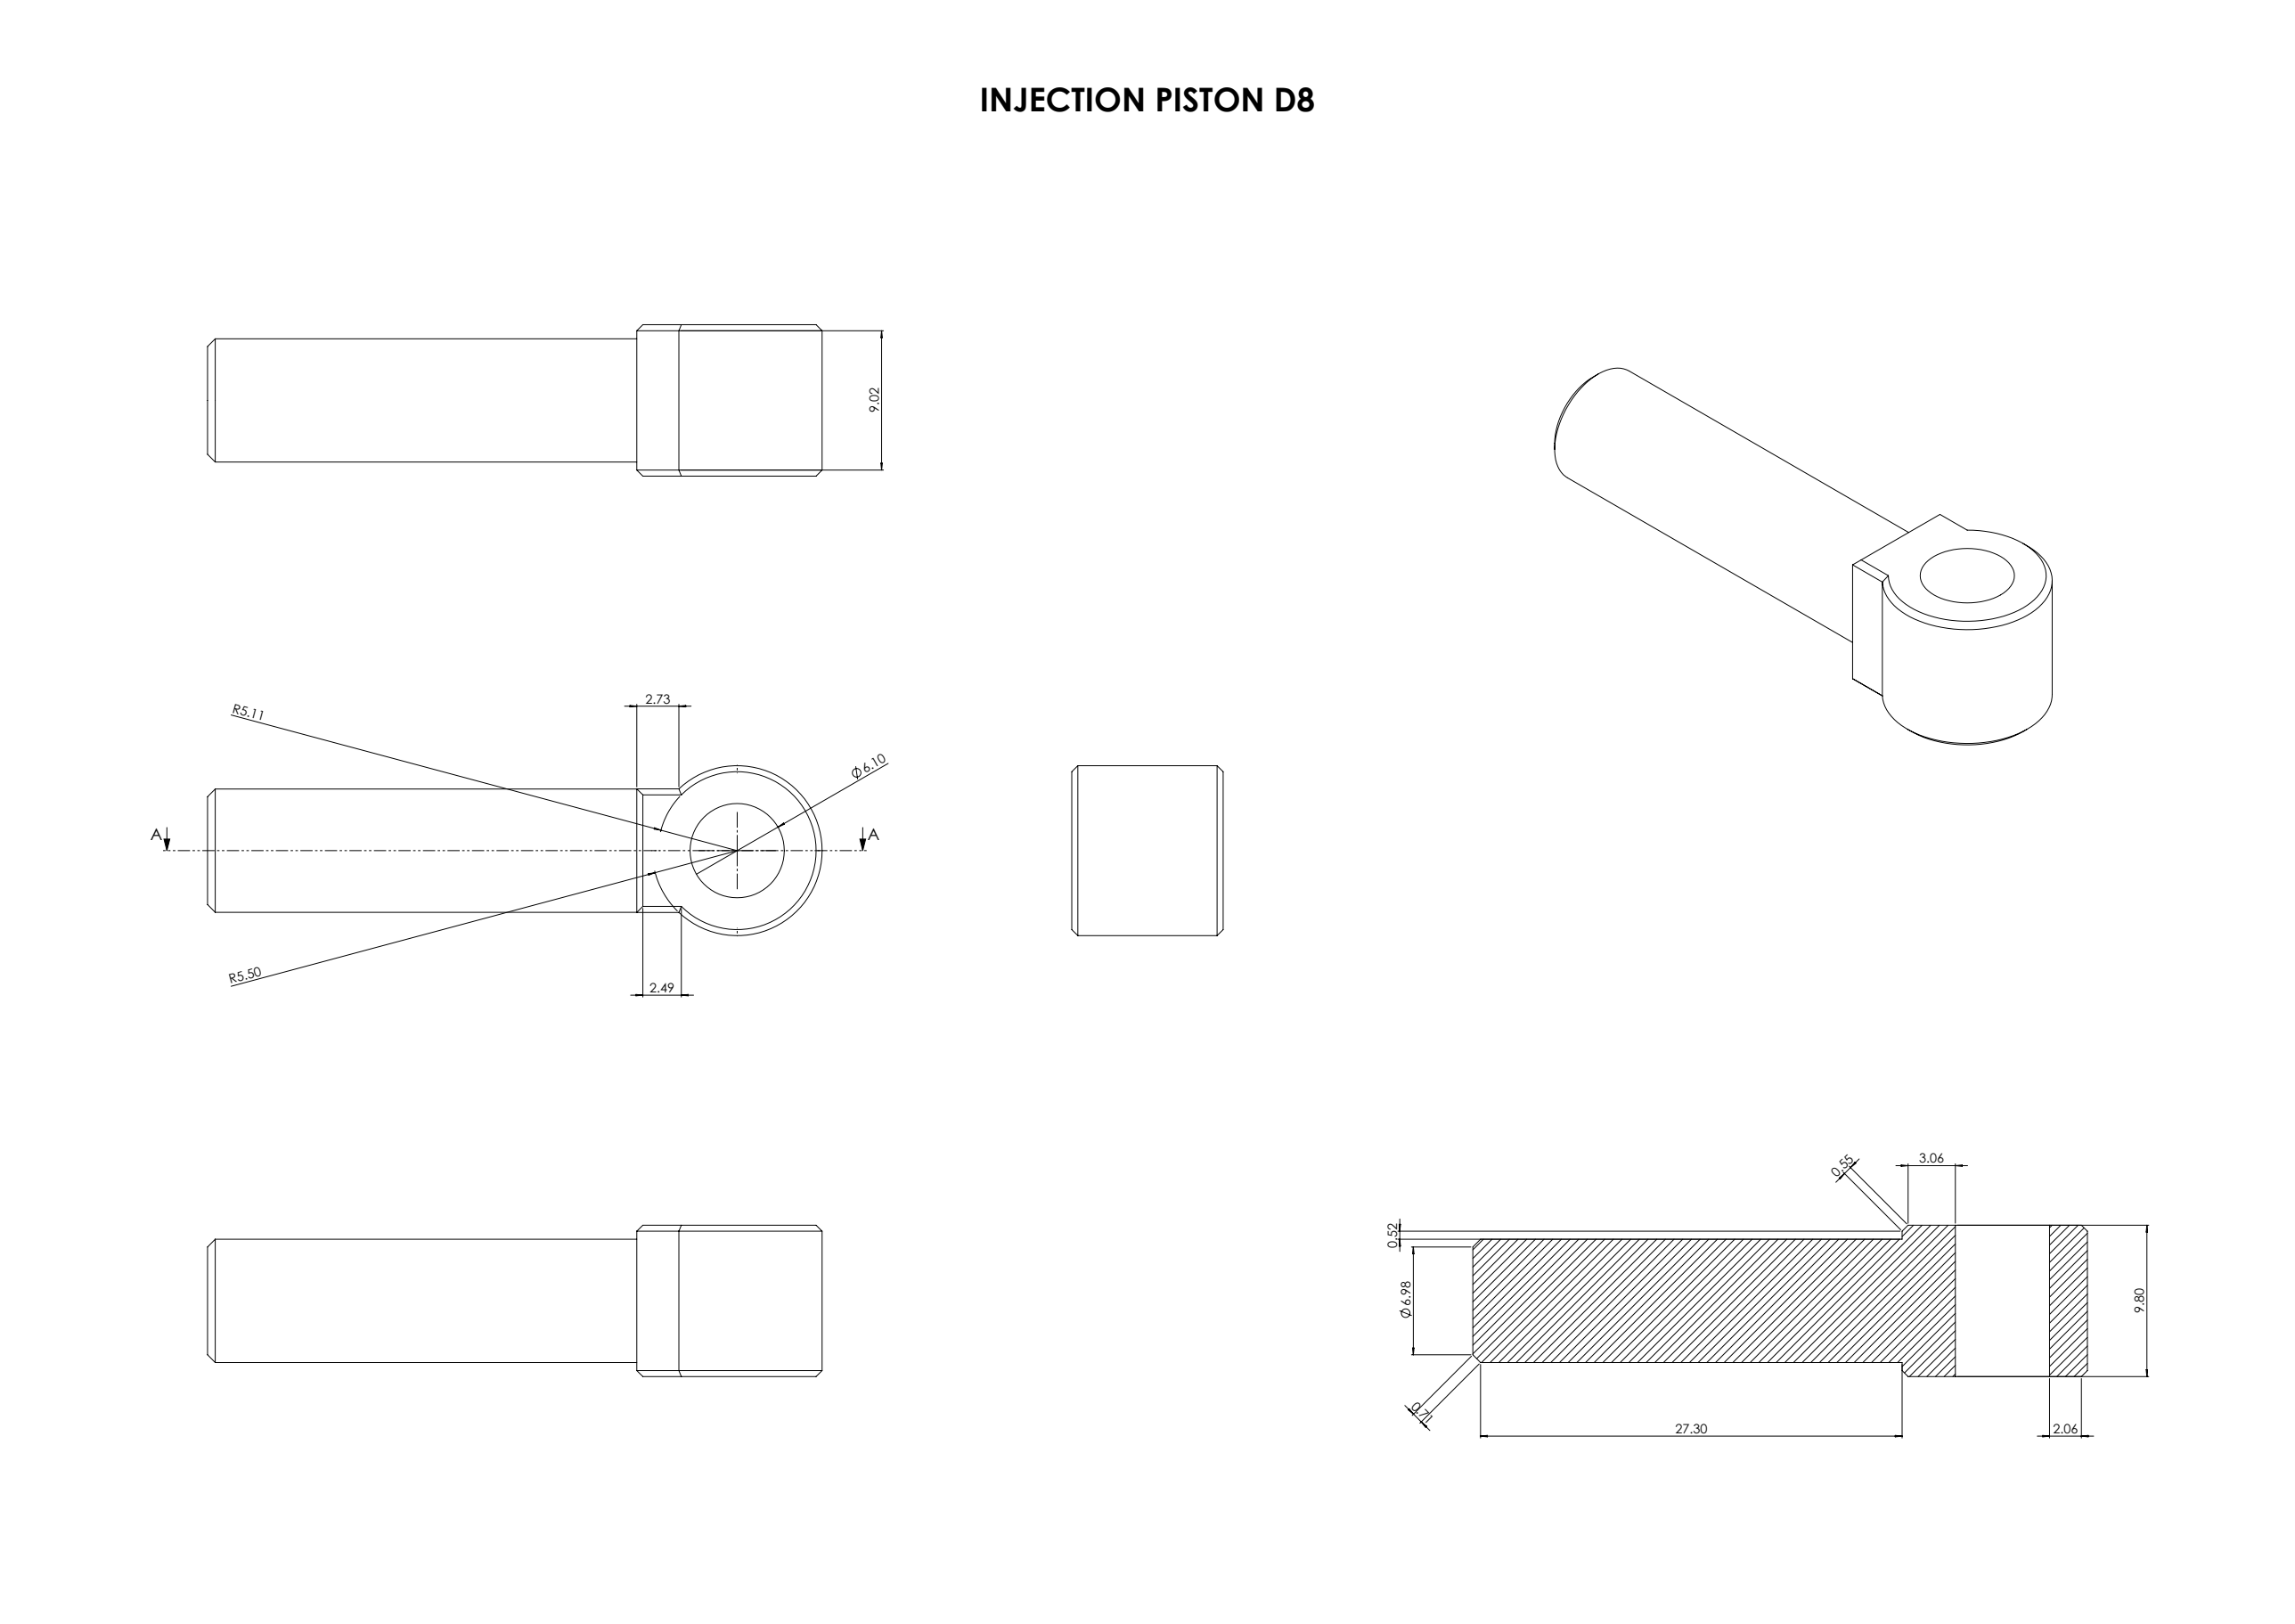
ISO-10303-21;
HEADER;
/* Generated by software containing ST-Developer
 * from STEP Tools, Inc. (www.steptools.com) 
 */

FILE_DESCRIPTION(
/* description */ (''),
/* implementation_level */ '2;1');

FILE_NAME(
/* name */ '13_Injection_Piston_D8.step',
/* time_stamp */ '2026-10-26T03:55:20-07:00',
/* author */ (''),
/* organization */ (''),
/* preprocessor_version */ 'ST-DEVELOPER v20.2',
/* originating_system */ 'Autodesk Translation Framework v15.15.0.0',
/* authorisation */ '');

FILE_SCHEMA (('AUTOMOTIVE_DESIGN { 1 0 10303 214 3 1 1 }'));
ENDSEC;

DATA;
#10=MECHANICAL_DESIGN_GEOMETRIC_PRESENTATION_REPRESENTATION('',(#193),#45236);
#153=SHAPE_REPRESENTATION_RELATIONSHIP('SRR','None',#45332,#173);
#173=ADVANCED_BREP_SHAPE_REPRESENTATION('',(#213),#45234);
#193=STYLED_ITEM('',(#45477),#213);
#213=MANIFOLD_SOLID_BREP('Body1',#16535);
#810=B_SPLINE_CURVE_WITH_KNOTS('',3,(#45054,#45055,#45056,#45057),
 .UNSPECIFIED.,.F.,.F.,(4,4),(-0.0573534079505418,0.),.UNSPECIFIED.);
#811=B_SPLINE_CURVE_WITH_KNOTS('',3,(#45060,#45061,#45062,#45063),
 .UNSPECIFIED.,.F.,.F.,(4,4),(-0.0573534079505118,0.),.UNSPECIFIED.);
#812=B_SPLINE_CURVE_WITH_KNOTS('',3,(#45094,#45095,#45096,#45097),
 .UNSPECIFIED.,.F.,.F.,(4,4),(-0.0573537350950076,0.),.UNSPECIFIED.);
#813=B_SPLINE_CURVE_WITH_KNOTS('',3,(#45100,#45101,#45102,#45103),
 .UNSPECIFIED.,.F.,.F.,(4,4),(-0.0573534079504966,0.),.UNSPECIFIED.);
#1059=FACE_BOUND('',#3866,.T.);
#1060=FACE_BOUND('',#3873,.T.);
#1061=FACE_BOUND('',#3876,.T.);
#1547=PLANE('',#18058);
#1548=PLANE('',#18059);
#1549=PLANE('',#18060);
#1550=PLANE('',#18061);
#1551=PLANE('',#18064);
#1552=PLANE('',#18068);
#1553=PLANE('',#18069);
#1554=PLANE('',#18070);
#1555=PLANE('',#18071);
#1556=PLANE('',#18072);
#1557=PLANE('',#18075);
#1558=PLANE('',#18077);
#1810=CYLINDRICAL_SURFACE('',#18062,5.5);
#1811=CYLINDRICAL_SURFACE('',#18074,3.05);
#1812=CYLINDRICAL_SURFACE('',#18081,3.99);
#2765=FACE_OUTER_BOUND('',#3859,.T.);
#2766=FACE_OUTER_BOUND('',#3860,.T.);
#2767=FACE_OUTER_BOUND('',#3861,.T.);
#2768=FACE_OUTER_BOUND('',#3862,.T.);
#2769=FACE_OUTER_BOUND('',#3863,.T.);
#2770=FACE_OUTER_BOUND('',#3864,.T.);
#2771=FACE_OUTER_BOUND('',#3865,.T.);
#2772=FACE_OUTER_BOUND('',#3867,.T.);
#2773=FACE_OUTER_BOUND('',#3868,.T.);
#2774=FACE_OUTER_BOUND('',#3869,.T.);
#2775=FACE_OUTER_BOUND('',#3870,.T.);
#2776=FACE_OUTER_BOUND('',#3871,.T.);
#2777=FACE_OUTER_BOUND('',#3872,.T.);
#2778=FACE_OUTER_BOUND('',#3874,.T.);
#2779=FACE_OUTER_BOUND('',#3875,.T.);
#2780=FACE_OUTER_BOUND('',#3877,.T.);
#2781=FACE_OUTER_BOUND('',#3878,.T.);
#2782=FACE_OUTER_BOUND('',#3879,.T.);
#3859=EDGE_LOOP('',(#15382,#15383,#15384,#15385));
#3860=EDGE_LOOP('',(#15386,#15387,#15388,#15389));
#3861=EDGE_LOOP('',(#15390,#15391,#15392,#15393));
#3862=EDGE_LOOP('',(#15394,#15395,#15396,#15397));
#3863=EDGE_LOOP('',(#15398,#15399,#15400,#15401));
#3864=EDGE_LOOP('',(#15402,#15403,#15404,#15405));
#3865=EDGE_LOOP('',(#15406,#15407,#15408,#15409));
#3866=EDGE_LOOP('',(#15410));
#3867=EDGE_LOOP('',(#15411,#15412,#15413,#15414));
#3868=EDGE_LOOP('',(#15415,#15416,#15417,#15418));
#3869=EDGE_LOOP('',(#15419,#15420,#15421,#15422));
#3870=EDGE_LOOP('',(#15423,#15424,#15425,#15426));
#3871=EDGE_LOOP('',(#15427,#15428,#15429,#15430));
#3872=EDGE_LOOP('',(#15431,#15432,#15433,#15434));
#3873=EDGE_LOOP('',(#15435));
#3874=EDGE_LOOP('',(#15436,#15437,#15438,#15439));
#3875=EDGE_LOOP('',(#15440,#15441,#15442,#15443));
#3876=EDGE_LOOP('',(#15444));
#3877=EDGE_LOOP('',(#15445));
#3878=EDGE_LOOP('',(#15446,#15447,#15448,#15449));
#3879=EDGE_LOOP('',(#15450,#15451,#15452,#15453));
#5166=LINE('',#45066,#6477);
#5167=LINE('',#45068,#6478);
#5168=LINE('',#45069,#6479);
#5169=LINE('',#45072,#6480);
#5170=LINE('',#45074,#6481);
#5171=LINE('',#45075,#6482);
#5172=LINE('',#45077,#6483);
#5173=LINE('',#45078,#6484);
#5174=LINE('',#45081,#6485);
#5175=LINE('',#45083,#6486);
#5176=LINE('',#45084,#6487);
#5177=LINE('',#45087,#6488);
#5178=LINE('',#45106,#6489);
#5179=LINE('',#45107,#6490);
#5180=LINE('',#45110,#6491);
#5181=LINE('',#45112,#6492);
#5182=LINE('',#45113,#6493);
#5183=LINE('',#45115,#6494);
#5184=LINE('',#45116,#6495);
#5185=LINE('',#45118,#6496);
#5186=LINE('',#45123,#6497);
#5187=LINE('',#45133,#6498);
#5188=LINE('',#45135,#6499);
#6477=VECTOR('',#22005,10.);
#6478=VECTOR('',#22006,10.);
#6479=VECTOR('',#22007,10.);
#6480=VECTOR('',#22010,10.);
#6481=VECTOR('',#22011,10.);
#6482=VECTOR('',#22012,10.);
#6483=VECTOR('',#22015,10.);
#6484=VECTOR('',#22016,10.);
#6485=VECTOR('',#22019,10.);
#6486=VECTOR('',#22020,10.);
#6487=VECTOR('',#22021,10.);
#6488=VECTOR('',#22024,10.);
#6489=VECTOR('',#22037,10.);
#6490=VECTOR('',#22038,10.);
#6491=VECTOR('',#22041,10.);
#6492=VECTOR('',#22042,10.);
#6493=VECTOR('',#22043,10.);
#6494=VECTOR('',#22046,10.);
#6495=VECTOR('',#22047,10.);
#6496=VECTOR('',#22050,10.);
#6497=VECTOR('',#22057,3.05);
#6498=VECTOR('',#22070,3.74);
#6499=VECTOR('',#22073,3.99);
#6950=CIRCLE('',#18056,5.11);
#6951=CIRCLE('',#18057,5.5);
#6952=CIRCLE('',#18063,5.5);
#6953=CIRCLE('',#18065,3.05);
#6954=CIRCLE('',#18067,5.11);
#6955=CIRCLE('',#18073,3.05);
#6956=CIRCLE('',#18076,3.99);
#6957=CIRCLE('',#18078,3.49);
#6958=CIRCLE('',#18080,3.99);
#8435=VERTEX_POINT('',#45050);
#8436=VERTEX_POINT('',#45051);
#8437=VERTEX_POINT('',#45053);
#8438=VERTEX_POINT('',#45058);
#8439=VERTEX_POINT('',#45065);
#8440=VERTEX_POINT('',#45067);
#8441=VERTEX_POINT('',#45071);
#8442=VERTEX_POINT('',#45073);
#8443=VERTEX_POINT('',#45080);
#8444=VERTEX_POINT('',#45082);
#8445=VERTEX_POINT('',#45086);
#8446=VERTEX_POINT('',#45090);
#8447=VERTEX_POINT('',#45093);
#8448=VERTEX_POINT('',#45098);
#8449=VERTEX_POINT('',#45105);
#8450=VERTEX_POINT('',#45109);
#8451=VERTEX_POINT('',#45111);
#8452=VERTEX_POINT('',#45120);
#8453=VERTEX_POINT('',#45125);
#8454=VERTEX_POINT('',#45128);
#8455=VERTEX_POINT('',#45131);
#10754=EDGE_CURVE('',#8435,#8436,#6950,.T.);
#10755=EDGE_CURVE('',#8436,#8437,#810,.T.);
#10756=EDGE_CURVE('',#8437,#8438,#6951,.T.);
#10757=EDGE_CURVE('',#8435,#8438,#811,.T.);
#10758=EDGE_CURVE('',#8436,#8439,#5166,.T.);
#10759=EDGE_CURVE('',#8439,#8440,#5167,.T.);
#10760=EDGE_CURVE('',#8440,#8437,#5168,.T.);
#10761=EDGE_CURVE('',#8439,#8441,#5169,.T.);
#10762=EDGE_CURVE('',#8441,#8442,#5170,.T.);
#10763=EDGE_CURVE('',#8442,#8440,#5171,.T.);
#10764=EDGE_CURVE('',#8438,#8442,#5172,.T.);
#10765=EDGE_CURVE('',#8441,#8435,#5173,.T.);
#10766=EDGE_CURVE('',#8443,#8438,#5174,.T.);
#10767=EDGE_CURVE('',#8444,#8443,#5175,.T.);
#10768=EDGE_CURVE('',#8444,#8442,#5176,.T.);
#10769=EDGE_CURVE('',#8445,#8437,#5177,.T.);
#10770=EDGE_CURVE('',#8443,#8445,#6952,.T.);
#10771=EDGE_CURVE('',#8446,#8446,#6953,.T.);
#10772=EDGE_CURVE('',#8445,#8447,#812,.T.);
#10773=EDGE_CURVE('',#8447,#8448,#6954,.T.);
#10774=EDGE_CURVE('',#8448,#8443,#813,.T.);
#10775=EDGE_CURVE('',#8448,#8449,#5178,.T.);
#10776=EDGE_CURVE('',#8449,#8444,#5179,.T.);
#10777=EDGE_CURVE('',#8449,#8450,#5180,.T.);
#10778=EDGE_CURVE('',#8450,#8451,#5181,.T.);
#10779=EDGE_CURVE('',#8451,#8444,#5182,.T.);
#10780=EDGE_CURVE('',#8445,#8451,#5183,.T.);
#10781=EDGE_CURVE('',#8450,#8447,#5184,.T.);
#10782=EDGE_CURVE('',#8451,#8440,#5185,.T.);
#10783=EDGE_CURVE('',#8452,#8452,#6955,.T.);
#10784=EDGE_CURVE('',#8452,#8446,#5186,.T.);
#10785=EDGE_CURVE('',#8453,#8453,#6956,.T.);
#10786=EDGE_CURVE('',#8454,#8454,#6957,.T.);
#10787=EDGE_CURVE('',#8455,#8455,#6958,.T.);
#10788=EDGE_CURVE('',#8455,#8454,#5187,.T.);
#10789=EDGE_CURVE('',#8453,#8455,#5188,.T.);
#15382=ORIENTED_EDGE('',*,*,#10754,.T.);
#15383=ORIENTED_EDGE('',*,*,#10755,.T.);
#15384=ORIENTED_EDGE('',*,*,#10756,.T.);
#15385=ORIENTED_EDGE('',*,*,#10757,.F.);
#15386=ORIENTED_EDGE('',*,*,#10758,.T.);
#15387=ORIENTED_EDGE('',*,*,#10759,.T.);
#15388=ORIENTED_EDGE('',*,*,#10760,.T.);
#15389=ORIENTED_EDGE('',*,*,#10755,.F.);
#15390=ORIENTED_EDGE('',*,*,#10761,.T.);
#15391=ORIENTED_EDGE('',*,*,#10762,.T.);
#15392=ORIENTED_EDGE('',*,*,#10763,.T.);
#15393=ORIENTED_EDGE('',*,*,#10759,.F.);
#15394=ORIENTED_EDGE('',*,*,#10764,.T.);
#15395=ORIENTED_EDGE('',*,*,#10762,.F.);
#15396=ORIENTED_EDGE('',*,*,#10765,.T.);
#15397=ORIENTED_EDGE('',*,*,#10757,.T.);
#15398=ORIENTED_EDGE('',*,*,#10764,.F.);
#15399=ORIENTED_EDGE('',*,*,#10766,.F.);
#15400=ORIENTED_EDGE('',*,*,#10767,.F.);
#15401=ORIENTED_EDGE('',*,*,#10768,.T.);
#15402=ORIENTED_EDGE('',*,*,#10756,.F.);
#15403=ORIENTED_EDGE('',*,*,#10769,.F.);
#15404=ORIENTED_EDGE('',*,*,#10770,.F.);
#15405=ORIENTED_EDGE('',*,*,#10766,.T.);
#15406=ORIENTED_EDGE('',*,*,#10754,.F.);
#15407=ORIENTED_EDGE('',*,*,#10765,.F.);
#15408=ORIENTED_EDGE('',*,*,#10761,.F.);
#15409=ORIENTED_EDGE('',*,*,#10758,.F.);
#15410=ORIENTED_EDGE('',*,*,#10771,.T.);
#15411=ORIENTED_EDGE('',*,*,#10770,.T.);
#15412=ORIENTED_EDGE('',*,*,#10772,.T.);
#15413=ORIENTED_EDGE('',*,*,#10773,.T.);
#15414=ORIENTED_EDGE('',*,*,#10774,.T.);
#15415=ORIENTED_EDGE('',*,*,#10775,.T.);
#15416=ORIENTED_EDGE('',*,*,#10776,.T.);
#15417=ORIENTED_EDGE('',*,*,#10767,.T.);
#15418=ORIENTED_EDGE('',*,*,#10774,.F.);
#15419=ORIENTED_EDGE('',*,*,#10777,.T.);
#15420=ORIENTED_EDGE('',*,*,#10778,.T.);
#15421=ORIENTED_EDGE('',*,*,#10779,.T.);
#15422=ORIENTED_EDGE('',*,*,#10776,.F.);
#15423=ORIENTED_EDGE('',*,*,#10780,.T.);
#15424=ORIENTED_EDGE('',*,*,#10778,.F.);
#15425=ORIENTED_EDGE('',*,*,#10781,.T.);
#15426=ORIENTED_EDGE('',*,*,#10772,.F.);
#15427=ORIENTED_EDGE('',*,*,#10760,.F.);
#15428=ORIENTED_EDGE('',*,*,#10782,.F.);
#15429=ORIENTED_EDGE('',*,*,#10780,.F.);
#15430=ORIENTED_EDGE('',*,*,#10769,.T.);
#15431=ORIENTED_EDGE('',*,*,#10773,.F.);
#15432=ORIENTED_EDGE('',*,*,#10781,.F.);
#15433=ORIENTED_EDGE('',*,*,#10777,.F.);
#15434=ORIENTED_EDGE('',*,*,#10775,.F.);
#15435=ORIENTED_EDGE('',*,*,#10783,.T.);
#15436=ORIENTED_EDGE('',*,*,#10783,.F.);
#15437=ORIENTED_EDGE('',*,*,#10784,.T.);
#15438=ORIENTED_EDGE('',*,*,#10771,.F.);
#15439=ORIENTED_EDGE('',*,*,#10784,.F.);
#15440=ORIENTED_EDGE('',*,*,#10763,.F.);
#15441=ORIENTED_EDGE('',*,*,#10768,.F.);
#15442=ORIENTED_EDGE('',*,*,#10779,.F.);
#15443=ORIENTED_EDGE('',*,*,#10782,.T.);
#15444=ORIENTED_EDGE('',*,*,#10785,.F.);
#15445=ORIENTED_EDGE('',*,*,#10786,.F.);
#15446=ORIENTED_EDGE('',*,*,#10787,.F.);
#15447=ORIENTED_EDGE('',*,*,#10788,.T.);
#15448=ORIENTED_EDGE('',*,*,#10786,.T.);
#15449=ORIENTED_EDGE('',*,*,#10788,.F.);
#15450=ORIENTED_EDGE('',*,*,#10785,.T.);
#15451=ORIENTED_EDGE('',*,*,#10789,.T.);
#15452=ORIENTED_EDGE('',*,*,#10787,.T.);
#15453=ORIENTED_EDGE('',*,*,#10789,.F.);
#15540=CONICAL_SURFACE('',#18055,5.305,0.785398163397448);
#15541=CONICAL_SURFACE('',#18066,5.305,0.785398163397449);
#15542=CONICAL_SURFACE('',#18079,3.74,0.78539816339745);
#16493=ADVANCED_FACE('',(#2765),#15540,.T.);
#16494=ADVANCED_FACE('',(#2766),#1547,.T.);
#16495=ADVANCED_FACE('',(#2767),#1548,.T.);
#16496=ADVANCED_FACE('',(#2768),#1549,.T.);
#16497=ADVANCED_FACE('',(#2769),#1550,.T.);
#16498=ADVANCED_FACE('',(#2770),#1810,.T.);
#16499=ADVANCED_FACE('',(#2771,#1059),#1551,.T.);
#16500=ADVANCED_FACE('',(#2772),#15541,.T.);
#16501=ADVANCED_FACE('',(#2773),#1552,.T.);
#16502=ADVANCED_FACE('',(#2774),#1553,.T.);
#16503=ADVANCED_FACE('',(#2775),#1554,.T.);
#16504=ADVANCED_FACE('',(#2776),#1555,.T.);
#16505=ADVANCED_FACE('',(#2777,#1060),#1556,.F.);
#16506=ADVANCED_FACE('',(#2778),#1811,.F.);
#16507=ADVANCED_FACE('',(#2779,#1061),#1557,.T.);
#16508=ADVANCED_FACE('',(#2780),#1558,.T.);
#16509=ADVANCED_FACE('',(#2781),#15542,.T.);
#16510=ADVANCED_FACE('',(#2782),#1812,.T.);
#16535=CLOSED_SHELL('',(#16493,#16494,#16495,#16496,#16497,#16498,#16499,
#16500,#16501,#16502,#16503,#16504,#16505,#16506,#16507,#16508,#16509,#16510));
#18054=AXIS2_PLACEMENT_3D('',#45048,#21995,#21996);
#18055=AXIS2_PLACEMENT_3D('',#45049,#21997,#21998);
#18056=AXIS2_PLACEMENT_3D('',#45052,#21999,#22000);
#18057=AXIS2_PLACEMENT_3D('',#45059,#22001,#22002);
#18058=AXIS2_PLACEMENT_3D('',#45064,#22003,#22004);
#18059=AXIS2_PLACEMENT_3D('',#45070,#22008,#22009);
#18060=AXIS2_PLACEMENT_3D('',#45076,#22013,#22014);
#18061=AXIS2_PLACEMENT_3D('',#45079,#22017,#22018);
#18062=AXIS2_PLACEMENT_3D('',#45085,#22022,#22023);
#18063=AXIS2_PLACEMENT_3D('',#45088,#22025,#22026);
#18064=AXIS2_PLACEMENT_3D('',#45089,#22027,#22028);
#18065=AXIS2_PLACEMENT_3D('',#45091,#22029,#22030);
#18066=AXIS2_PLACEMENT_3D('',#45092,#22031,#22032);
#18067=AXIS2_PLACEMENT_3D('',#45099,#22033,#22034);
#18068=AXIS2_PLACEMENT_3D('',#45104,#22035,#22036);
#18069=AXIS2_PLACEMENT_3D('',#45108,#22039,#22040);
#18070=AXIS2_PLACEMENT_3D('',#45114,#22044,#22045);
#18071=AXIS2_PLACEMENT_3D('',#45117,#22048,#22049);
#18072=AXIS2_PLACEMENT_3D('',#45119,#22051,#22052);
#18073=AXIS2_PLACEMENT_3D('',#45121,#22053,#22054);
#18074=AXIS2_PLACEMENT_3D('',#45122,#22055,#22056);
#18075=AXIS2_PLACEMENT_3D('',#45124,#22058,#22059);
#18076=AXIS2_PLACEMENT_3D('',#45126,#22060,#22061);
#18077=AXIS2_PLACEMENT_3D('',#45127,#22062,#22063);
#18078=AXIS2_PLACEMENT_3D('',#45129,#22064,#22065);
#18079=AXIS2_PLACEMENT_3D('',#45130,#22066,#22067);
#18080=AXIS2_PLACEMENT_3D('',#45132,#22068,#22069);
#18081=AXIS2_PLACEMENT_3D('',#45134,#22071,#22072);
#21995=DIRECTION('axis',(0.,0.,1.));
#21996=DIRECTION('refdir',(1.,0.,0.));
#21997=DIRECTION('center_axis',(0.,-1.,0.));
#21998=DIRECTION('ref_axis',(1.,0.,0.));
#21999=DIRECTION('center_axis',(0.,-1.,0.));
#22000=DIRECTION('ref_axis',(1.,0.,0.));
#22001=DIRECTION('center_axis',(0.,1.,0.));
#22002=DIRECTION('ref_axis',(1.,0.,0.));
#22003=DIRECTION('center_axis',(0.,0.707106781186548,0.707106781186547));
#22004=DIRECTION('ref_axis',(1.,0.,0.));
#22005=DIRECTION('',(-1.,0.,0.));
#22006=DIRECTION('',(-0.577350269189626,-0.577350269189626,0.577350269189626));
#22007=DIRECTION('',(1.,0.,0.));
#22008=DIRECTION('center_axis',(-0.707106781186547,0.707106781186548,0.));
#22009=DIRECTION('ref_axis',(0.,0.,1.));
#22010=DIRECTION('',(0.,0.,-1.));
#22011=DIRECTION('',(-0.577350269189626,-0.577350269189626,-0.577350269189626));
#22012=DIRECTION('',(0.,0.,1.));
#22013=DIRECTION('center_axis',(0.,0.707106781186548,-0.707106781186547));
#22014=DIRECTION('ref_axis',(-1.,0.,0.));
#22015=DIRECTION('',(-1.,0.,0.));
#22016=DIRECTION('',(1.,0.,0.));
#22017=DIRECTION('center_axis',(0.,0.,-1.));
#22018=DIRECTION('ref_axis',(-1.,0.,0.));
#22019=DIRECTION('',(0.,1.,0.));
#22020=DIRECTION('',(1.,0.,0.));
#22021=DIRECTION('',(0.,1.,0.));
#22022=DIRECTION('center_axis',(0.,1.,0.));
#22023=DIRECTION('ref_axis',(1.,0.,0.));
#22024=DIRECTION('',(0.,1.,0.));
#22025=DIRECTION('center_axis',(0.,-1.,0.));
#22026=DIRECTION('ref_axis',(1.,0.,0.));
#22027=DIRECTION('center_axis',(0.,1.,0.));
#22028=DIRECTION('ref_axis',(1.,0.,0.));
#22029=DIRECTION('center_axis',(0.,-1.,0.));
#22030=DIRECTION('ref_axis',(1.,0.,0.));
#22031=DIRECTION('center_axis',(0.,1.,0.));
#22032=DIRECTION('ref_axis',(1.,0.,0.));
#22033=DIRECTION('center_axis',(0.,1.,0.));
#22034=DIRECTION('ref_axis',(1.,0.,0.));
#22035=DIRECTION('center_axis',(0.,-0.707106781186548,-0.707106781186547));
#22036=DIRECTION('ref_axis',(-1.,0.,0.));
#22037=DIRECTION('',(-1.,0.,0.));
#22038=DIRECTION('',(-0.577350269189626,0.577350269189625,-0.577350269189626));
#22039=DIRECTION('center_axis',(-0.707106781186547,-0.707106781186548,0.));
#22040=DIRECTION('ref_axis',(0.,0.,1.));
#22041=DIRECTION('',(0.,0.,1.));
#22042=DIRECTION('',(-0.577350269189626,0.577350269189625,0.577350269189626));
#22043=DIRECTION('',(0.,0.,-1.));
#22044=DIRECTION('center_axis',(0.,-0.707106781186548,0.707106781186547));
#22045=DIRECTION('ref_axis',(1.,0.,0.));
#22046=DIRECTION('',(-1.,0.,0.));
#22047=DIRECTION('',(1.,0.,0.));
#22048=DIRECTION('center_axis',(0.,0.,1.));
#22049=DIRECTION('ref_axis',(1.,0.,0.));
#22050=DIRECTION('',(0.,1.,0.));
#22051=DIRECTION('center_axis',(0.,1.,0.));
#22052=DIRECTION('ref_axis',(1.,0.,0.));
#22053=DIRECTION('center_axis',(0.,1.,0.));
#22054=DIRECTION('ref_axis',(1.,0.,0.));
#22055=DIRECTION('center_axis',(0.,1.,0.));
#22056=DIRECTION('ref_axis',(1.,0.,0.));
#22057=DIRECTION('',(0.,1.,0.));
#22058=DIRECTION('center_axis',(-1.,0.,0.));
#22059=DIRECTION('ref_axis',(0.,0.,1.));
#22060=DIRECTION('center_axis',(-1.,0.,0.));
#22061=DIRECTION('ref_axis',(0.,1.,0.));
#22062=DIRECTION('center_axis',(-1.,0.,0.));
#22063=DIRECTION('ref_axis',(0.,0.,1.));
#22064=DIRECTION('center_axis',(1.,0.,0.));
#22065=DIRECTION('ref_axis',(0.,0.,-1.));
#22066=DIRECTION('center_axis',(1.,0.,0.));
#22067=DIRECTION('ref_axis',(0.,1.,0.));
#22068=DIRECTION('center_axis',(1.,0.,0.));
#22069=DIRECTION('ref_axis',(0.,0.,-1.));
#22070=DIRECTION('',(-0.707106781186546,0.707106781186549,8.65956056235495E-17));
#22071=DIRECTION('center_axis',(1.,0.,0.));
#22072=DIRECTION('ref_axis',(0.,1.,0.));
#22073=DIRECTION('',(-1.,0.,0.));
#45048=CARTESIAN_POINT('',(0.,0.,0.));
#45049=CARTESIAN_POINT('Origin',(0.,4.705,0.));
#45050=CARTESIAN_POINT('',(-3.61662826400503,4.9,-3.61));
#45051=CARTESIAN_POINT('',(-3.61662826400503,4.9,3.61));
#45052=CARTESIAN_POINT('Origin',(0.,4.9,0.));
#45053=CARTESIAN_POINT('',(-3.77491721763537,4.51,4.));
#45054=CARTESIAN_POINT('Ctrl Pts',(-3.61662826400502,4.9,3.61));
#45055=CARTESIAN_POINT('Ctrl Pts',(-3.67042997577938,4.77027947236335,3.73972052763665));
#45056=CARTESIAN_POINT('Ctrl Pts',(-3.72320339124168,4.64014360909558,3.86985639090442));
#45057=CARTESIAN_POINT('Ctrl Pts',(-3.77491721763537,4.51,4.));
#45058=CARTESIAN_POINT('',(-3.77491721763537,4.51,-4.));
#45059=CARTESIAN_POINT('Origin',(0.,4.51,0.));
#45060=CARTESIAN_POINT('Ctrl Pts',(-3.61662826400502,4.9,-3.61));
#45061=CARTESIAN_POINT('Ctrl Pts',(-3.67042997577939,4.77027947236332,-3.73972052763668));
#45062=CARTESIAN_POINT('Ctrl Pts',(-3.7232033912417,4.64014360909552,-3.86985639090449));
#45063=CARTESIAN_POINT('Ctrl Pts',(-3.77491721763537,4.51,-4.));
#45064=CARTESIAN_POINT('Origin',(-3.5,4.705,3.805));
#45065=CARTESIAN_POINT('',(-6.11,4.9,3.61));
#45066=CARTESIAN_POINT('',(-3.5,4.9,3.61));
#45067=CARTESIAN_POINT('',(-6.5,4.51,4.));
#45068=CARTESIAN_POINT('',(-6.11,4.9,3.61));
#45069=CARTESIAN_POINT('',(-3.5,4.51,4.));
#45070=CARTESIAN_POINT('Origin',(-6.305,4.705,-2.));
#45071=CARTESIAN_POINT('',(-6.11,4.9,-3.61));
#45072=CARTESIAN_POINT('',(-6.11,4.9,-2.));
#45073=CARTESIAN_POINT('',(-6.5,4.51,-4.));
#45074=CARTESIAN_POINT('',(-6.11,4.9,-3.61));
#45075=CARTESIAN_POINT('',(-6.5,4.51,-2.));
#45076=CARTESIAN_POINT('Origin',(-2.13745860881769,4.705,-3.805));
#45077=CARTESIAN_POINT('',(-2.13745860881769,4.51,-4.));
#45078=CARTESIAN_POINT('',(-2.13745860881769,4.9,-3.61));
#45079=CARTESIAN_POINT('Origin',(-3.77491721763537,-4.9,-4.));
#45080=CARTESIAN_POINT('',(-3.77491721763537,-4.51,-4.));
#45081=CARTESIAN_POINT('',(-3.77491721763537,-4.9,-4.));
#45082=CARTESIAN_POINT('',(-6.5,-4.51,-4.));
#45083=CARTESIAN_POINT('',(-2.13745860881769,-4.51,-4.));
#45084=CARTESIAN_POINT('',(-6.5,-4.9,-4.));
#45085=CARTESIAN_POINT('Origin',(0.,-4.9,0.));
#45086=CARTESIAN_POINT('',(-3.77491721763537,-4.51,4.));
#45087=CARTESIAN_POINT('',(-3.77491721763537,-4.9,4.));
#45088=CARTESIAN_POINT('Origin',(0.,-4.51,0.));
#45089=CARTESIAN_POINT('Origin',(-0.499999999999999,4.9,0.));
#45090=CARTESIAN_POINT('',(-3.05,4.9,-3.73517273739943E-16));
#45091=CARTESIAN_POINT('Origin',(0.,4.9,0.));
#45092=CARTESIAN_POINT('Origin',(0.,-4.705,0.));
#45093=CARTESIAN_POINT('',(-3.61662826400503,-4.9,3.61));
#45094=CARTESIAN_POINT('Ctrl Pts',(-3.77491721763537,-4.51,4.));
#45095=CARTESIAN_POINT('Ctrl Pts',(-3.72320339124172,-4.64014360909549,
3.86985639090451));
#45096=CARTESIAN_POINT('Ctrl Pts',(-3.6704299757794,-4.77027947236331,3.73972052763669));
#45097=CARTESIAN_POINT('Ctrl Pts',(-3.61662826400502,-4.9,3.61));
#45098=CARTESIAN_POINT('',(-3.61662826400503,-4.9,-3.61));
#45099=CARTESIAN_POINT('Origin',(0.,-4.9,0.));
#45100=CARTESIAN_POINT('Ctrl Pts',(-3.61662826400502,-4.9,-3.61));
#45101=CARTESIAN_POINT('Ctrl Pts',(-3.6704299757794,-4.77027947236331,-3.73972052763669));
#45102=CARTESIAN_POINT('Ctrl Pts',(-3.72320339124172,-4.64014360909548,
-3.86985639090452));
#45103=CARTESIAN_POINT('Ctrl Pts',(-3.77491721763537,-4.51,-4.));
#45104=CARTESIAN_POINT('Origin',(-2.13745860881769,-4.705,-3.805));
#45105=CARTESIAN_POINT('',(-6.11,-4.9,-3.61));
#45106=CARTESIAN_POINT('',(-2.13745860881769,-4.9,-3.61));
#45107=CARTESIAN_POINT('',(-6.11,-4.9,-3.61));
#45108=CARTESIAN_POINT('Origin',(-6.305,-4.705,-2.));
#45109=CARTESIAN_POINT('',(-6.11,-4.9,3.61));
#45110=CARTESIAN_POINT('',(-6.11,-4.9,-2.));
#45111=CARTESIAN_POINT('',(-6.5,-4.51,4.));
#45112=CARTESIAN_POINT('',(-6.11,-4.9,3.61));
#45113=CARTESIAN_POINT('',(-6.5,-4.51,-2.));
#45114=CARTESIAN_POINT('Origin',(-3.5,-4.705,3.805));
#45115=CARTESIAN_POINT('',(-3.5,-4.51,4.));
#45116=CARTESIAN_POINT('',(-3.5,-4.9,3.61));
#45117=CARTESIAN_POINT('Origin',(-6.5,-4.9,4.));
#45118=CARTESIAN_POINT('',(-6.5,-4.9,4.));
#45119=CARTESIAN_POINT('Origin',(-0.499999999999999,-4.9,0.));
#45120=CARTESIAN_POINT('',(-3.05,-4.9,3.73517273739943E-16));
#45121=CARTESIAN_POINT('Origin',(0.,-4.9,0.));
#45122=CARTESIAN_POINT('Origin',(0.,-5.,0.));
#45123=CARTESIAN_POINT('',(-3.05,-5.,3.73517273739943E-16));
#45124=CARTESIAN_POINT('Origin',(-6.5,-4.9,-4.));
#45125=CARTESIAN_POINT('',(-6.5,-3.99,4.88634072859794E-16));
#45126=CARTESIAN_POINT('Origin',(-6.5,0.,0.));
#45127=CARTESIAN_POINT('Origin',(-34.3,3.49,0.));
#45128=CARTESIAN_POINT('',(-34.3,-3.49,-4.27401732902426E-16));
#45129=CARTESIAN_POINT('Origin',(-34.3,0.,0.));
#45130=CARTESIAN_POINT('Origin',(-34.05,0.,0.));
#45131=CARTESIAN_POINT('',(-33.8,-3.99,-4.88634072859794E-16));
#45132=CARTESIAN_POINT('Origin',(-33.8,0.,0.));
#45133=CARTESIAN_POINT('',(-34.05,-3.74,-4.5801790288111E-16));
#45134=CARTESIAN_POINT('Origin',(-19.4,0.,0.));
#45135=CARTESIAN_POINT('',(-19.4,-3.99,-4.88634072859794E-16));
#45212=UNCERTAINTY_MEASURE_WITH_UNIT(LENGTH_MEASURE(0.01),#45237,
'DISTANCE_ACCURACY_VALUE',
'Maximum model space distance between geometric entities at asserted c
onnectivities');
#45214=UNCERTAINTY_MEASURE_WITH_UNIT(LENGTH_MEASURE(0.01),#45237,
'DISTANCE_ACCURACY_VALUE',
'Maximum model space distance between geometric entities at asserted c
onnectivities');
#45234=(
GEOMETRIC_REPRESENTATION_CONTEXT(3)
GLOBAL_UNCERTAINTY_ASSIGNED_CONTEXT((#45212))
GLOBAL_UNIT_ASSIGNED_CONTEXT((#45237,#45239,#45240))
REPRESENTATION_CONTEXT('','3D')
);
#45236=(
GEOMETRIC_REPRESENTATION_CONTEXT(3)
GLOBAL_UNCERTAINTY_ASSIGNED_CONTEXT((#45214))
GLOBAL_UNIT_ASSIGNED_CONTEXT((#45237,#45239,#45240))
REPRESENTATION_CONTEXT('','3D')
);
#45237=(
LENGTH_UNIT()
NAMED_UNIT(*)
SI_UNIT(.MILLI.,.METRE.)
);
#45239=(
NAMED_UNIT(*)
PLANE_ANGLE_UNIT()
SI_UNIT($,.RADIAN.)
);
#45240=(
NAMED_UNIT(*)
SI_UNIT($,.STERADIAN.)
SOLID_ANGLE_UNIT()
);
#45260=SHAPE_DEFINITION_REPRESENTATION(#45281,#45332);
#45281=PRODUCT_DEFINITION_SHAPE('',$,#45354);
#45332=SHAPE_REPRESENTATION('',(#18054),#45234);
#45334=PRODUCT_DEFINITION_CONTEXT('part definition',#45399,'design');
#45354=PRODUCT_DEFINITION('2026-10-25-23-38-21-279',
'13_Injection_Piston_D8',#45375,#45334);
#45375=PRODUCT_DEFINITION_FORMATION('',$,#45420);
#45399=APPLICATION_CONTEXT(
'Core Data for Automotive Mechanical Design Process');
#45400=PRODUCT_CONTEXT('part definition',#45399,'mechanical');
#45420=PRODUCT('2026-10-25-23-38-21-279','13_Injection_Piston_D8',$,(#45400));
#45471=COLOUR_RGB('Sky Blue',0.24,0.69,0.87);
#45472=FILL_AREA_STYLE_COLOUR('',#45471);
#45473=FILL_AREA_STYLE('',(#45472));
#45474=SURFACE_STYLE_FILL_AREA(#45473);
#45475=SURFACE_SIDE_STYLE('',(#45474));
#45476=SURFACE_STYLE_USAGE(.BOTH.,#45475);
#45477=PRESENTATION_STYLE_ASSIGNMENT((#45476));
ENDSEC;
END-ISO-10303-21;
